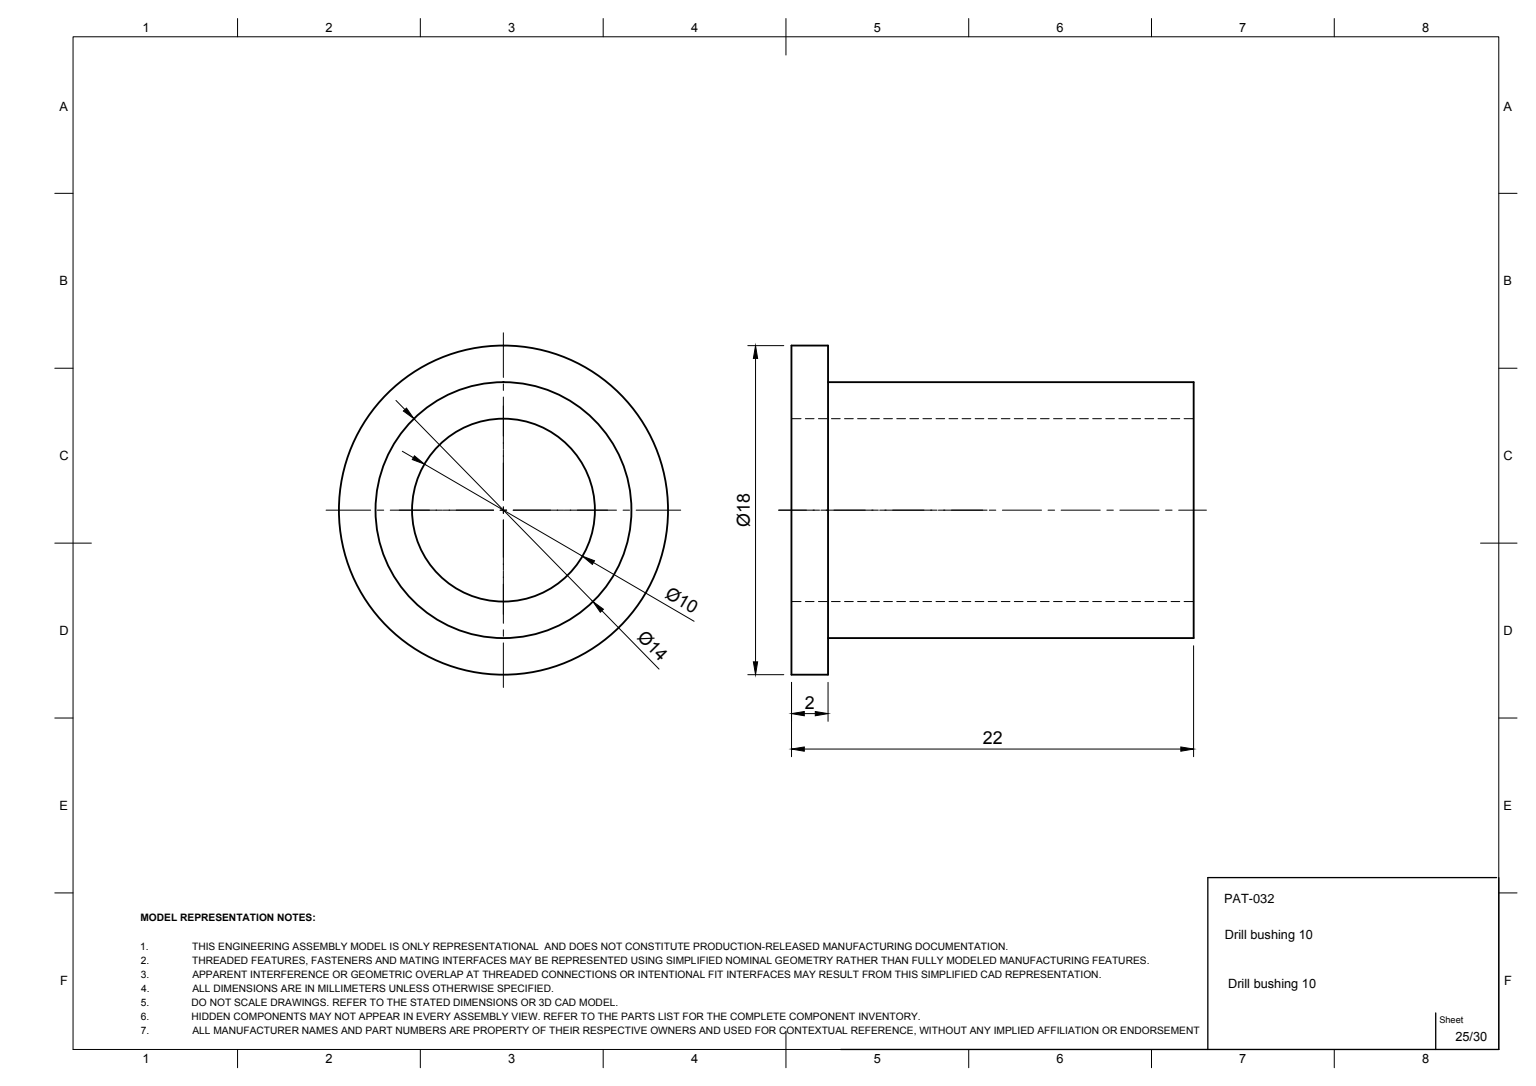
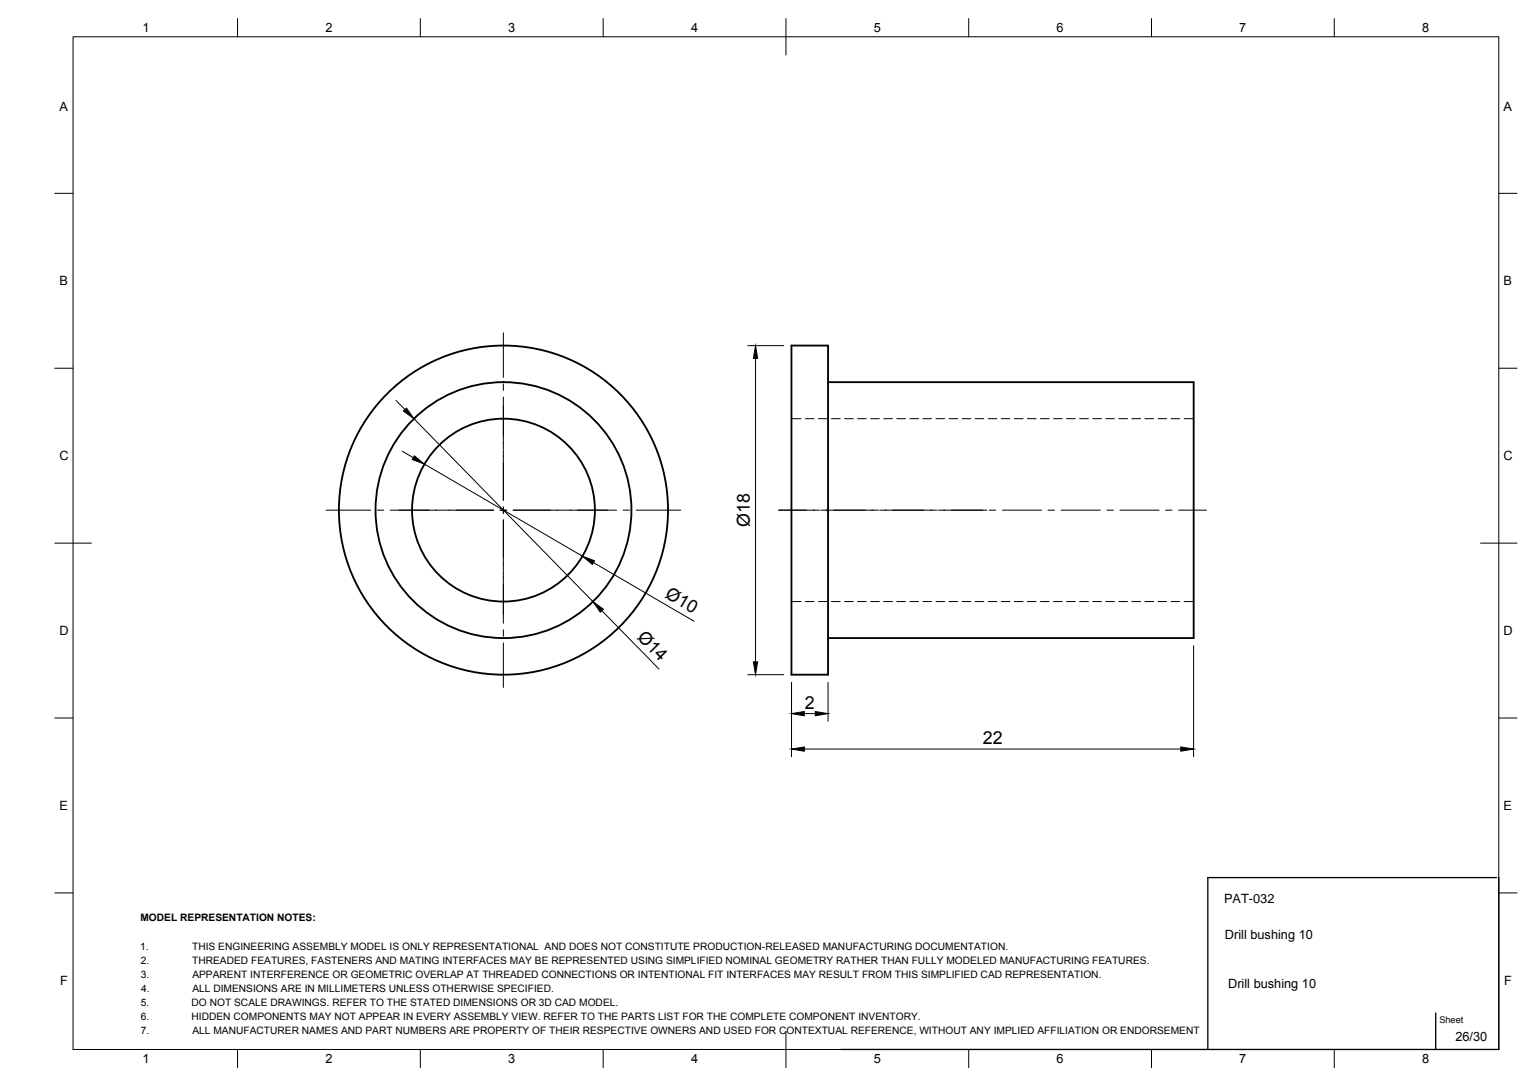
ISO-10303-21;
HEADER;
/* Generated by software containing ST-Developer
 * from STEP Tools, Inc. (www.steptools.com) 
 */

FILE_DESCRIPTION(
/* description */ ('Drill jig with bushing plate'),
/* implementation_level */ '2;1');

FILE_NAME(
/* name */ 'Drill bushing 10.step',
/* time_stamp */ '2026-10-27T10:51:08-07:00',
/* author */ (''),
/* organization */ (''),
/* preprocessor_version */ 'ST-DEVELOPER v20.2',
/* originating_system */ 'Autodesk Translation Framework v15.17.0.0',
/* authorisation */ '');

FILE_SCHEMA (('AUTOMOTIVE_DESIGN { 1 0 10303 214 3 1 1 }'));
ENDSEC;

DATA;
#10=MECHANICAL_DESIGN_GEOMETRIC_PRESENTATION_REPRESENTATION('',(#243),#6638);
#195=SHAPE_REPRESENTATION_RELATIONSHIP('SRR','None',#6760,#219);
#219=ADVANCED_BREP_SHAPE_REPRESENTATION('',(#265),#6633);
#243=STYLED_ITEM('',(#6929),#265);
#265=MANIFOLD_SOLID_BREP('Body1',#3612);
#361=FACE_BOUND('',#998,.T.);
#362=FACE_BOUND('',#1001,.T.);
#363=FACE_BOUND('',#1005,.T.);
#487=PLANE('',#4271);
#488=PLANE('',#4276);
#489=PLANE('',#4282);
#691=FACE_OUTER_BOUND('',#997,.T.);
#692=FACE_OUTER_BOUND('',#999,.T.);
#693=FACE_OUTER_BOUND('',#1000,.T.);
#694=FACE_OUTER_BOUND('',#1002,.T.);
#695=FACE_OUTER_BOUND('',#1003,.T.);
#696=FACE_OUTER_BOUND('',#1004,.T.);
#997=EDGE_LOOP('',(#3221));
#998=EDGE_LOOP('',(#3222));
#999=EDGE_LOOP('',(#3223,#3224,#3225,#3226));
#1000=EDGE_LOOP('',(#3227));
#1001=EDGE_LOOP('',(#3228));
#1002=EDGE_LOOP('',(#3229,#3230,#3231,#3232));
#1003=EDGE_LOOP('',(#3233,#3234,#3235,#3236));
#1004=EDGE_LOOP('',(#3237));
#1005=EDGE_LOOP('',(#3238));
#1272=LINE('',#6486,#1533);
#1273=LINE('',#6492,#1534);
#1274=LINE('',#6496,#1535);
#1533=VECTOR('',#5361,0.9);
#1534=VECTOR('',#5368,0.5);
#1535=VECTOR('',#5373,0.7);
#1700=CIRCLE('',#4272,0.9);
#1701=CIRCLE('',#4273,0.7);
#1702=CIRCLE('',#4275,0.9);
#1703=CIRCLE('',#4277,0.5);
#1704=CIRCLE('',#4279,0.5);
#1705=CIRCLE('',#4281,0.7);
#1980=VERTEX_POINT('',#6479);
#1981=VERTEX_POINT('',#6481);
#1982=VERTEX_POINT('',#6484);
#1983=VERTEX_POINT('',#6488);
#1984=VERTEX_POINT('',#6491);
#1985=VERTEX_POINT('',#6495);
#2398=EDGE_CURVE('',#1980,#1980,#1700,.T.);
#2399=EDGE_CURVE('',#1981,#1981,#1701,.T.);
#2400=EDGE_CURVE('',#1982,#1982,#1702,.T.);
#2401=EDGE_CURVE('',#1982,#1980,#1272,.T.);
#2402=EDGE_CURVE('',#1983,#1983,#1703,.T.);
#2403=EDGE_CURVE('',#1983,#1984,#1273,.T.);
#2404=EDGE_CURVE('',#1984,#1984,#1704,.T.);
#2405=EDGE_CURVE('',#1981,#1985,#1274,.T.);
#2406=EDGE_CURVE('',#1985,#1985,#1705,.T.);
#3221=ORIENTED_EDGE('',*,*,#2398,.F.);
#3222=ORIENTED_EDGE('',*,*,#2399,.T.);
#3223=ORIENTED_EDGE('',*,*,#2400,.F.);
#3224=ORIENTED_EDGE('',*,*,#2401,.T.);
#3225=ORIENTED_EDGE('',*,*,#2398,.T.);
#3226=ORIENTED_EDGE('',*,*,#2401,.F.);
#3227=ORIENTED_EDGE('',*,*,#2400,.T.);
#3228=ORIENTED_EDGE('',*,*,#2402,.T.);
#3229=ORIENTED_EDGE('',*,*,#2402,.F.);
#3230=ORIENTED_EDGE('',*,*,#2403,.T.);
#3231=ORIENTED_EDGE('',*,*,#2404,.T.);
#3232=ORIENTED_EDGE('',*,*,#2403,.F.);
#3233=ORIENTED_EDGE('',*,*,#2399,.F.);
#3234=ORIENTED_EDGE('',*,*,#2405,.T.);
#3235=ORIENTED_EDGE('',*,*,#2406,.T.);
#3236=ORIENTED_EDGE('',*,*,#2405,.F.);
#3237=ORIENTED_EDGE('',*,*,#2406,.F.);
#3238=ORIENTED_EDGE('',*,*,#2404,.F.);
#3366=CYLINDRICAL_SURFACE('',#4274,0.9);
#3367=CYLINDRICAL_SURFACE('',#4278,0.5);
#3368=CYLINDRICAL_SURFACE('',#4280,0.7);
#3566=ADVANCED_FACE('',(#691,#361),#487,.F.);
#3567=ADVANCED_FACE('',(#692),#3366,.T.);
#3568=ADVANCED_FACE('',(#693,#362),#488,.T.);
#3569=ADVANCED_FACE('',(#694),#3367,.F.);
#3570=ADVANCED_FACE('',(#695),#3368,.T.);
#3571=ADVANCED_FACE('',(#696,#363),#489,.F.);
#3612=CLOSED_SHELL('',(#3566,#3567,#3568,#3569,#3570,#3571));
#4270=AXIS2_PLACEMENT_3D('',#6477,#5349,#5350);
#4271=AXIS2_PLACEMENT_3D('',#6478,#5351,#5352);
#4272=AXIS2_PLACEMENT_3D('',#6480,#5353,#5354);
#4273=AXIS2_PLACEMENT_3D('',#6482,#5355,#5356);
#4274=AXIS2_PLACEMENT_3D('',#6483,#5357,#5358);
#4275=AXIS2_PLACEMENT_3D('',#6485,#5359,#5360);
#4276=AXIS2_PLACEMENT_3D('',#6487,#5362,#5363);
#4277=AXIS2_PLACEMENT_3D('',#6489,#5364,#5365);
#4278=AXIS2_PLACEMENT_3D('',#6490,#5366,#5367);
#4279=AXIS2_PLACEMENT_3D('',#6493,#5369,#5370);
#4280=AXIS2_PLACEMENT_3D('',#6494,#5371,#5372);
#4281=AXIS2_PLACEMENT_3D('',#6497,#5374,#5375);
#4282=AXIS2_PLACEMENT_3D('',#6498,#5376,#5377);
#5349=DIRECTION('axis',(0.,0.,1.));
#5350=DIRECTION('refdir',(1.,0.,0.));
#5351=DIRECTION('center_axis',(0.,0.,1.));
#5352=DIRECTION('ref_axis',(1.,0.,0.));
#5353=DIRECTION('center_axis',(0.,0.,1.));
#5354=DIRECTION('ref_axis',(1.,0.,0.));
#5355=DIRECTION('center_axis',(0.,0.,1.));
#5356=DIRECTION('ref_axis',(1.,0.,0.));
#5357=DIRECTION('center_axis',(0.,0.,1.));
#5358=DIRECTION('ref_axis',(1.,0.,0.));
#5359=DIRECTION('center_axis',(0.,0.,1.));
#5360=DIRECTION('ref_axis',(1.,0.,0.));
#5361=DIRECTION('',(0.,0.,-1.));
#5362=DIRECTION('center_axis',(0.,0.,1.));
#5363=DIRECTION('ref_axis',(1.,0.,0.));
#5364=DIRECTION('center_axis',(0.,0.,-1.));
#5365=DIRECTION('ref_axis',(1.,0.,0.));
#5366=DIRECTION('center_axis',(0.,0.,1.));
#5367=DIRECTION('ref_axis',(1.,0.,0.));
#5368=DIRECTION('',(0.,0.,-1.));
#5369=DIRECTION('center_axis',(0.,0.,-1.));
#5370=DIRECTION('ref_axis',(1.,0.,0.));
#5371=DIRECTION('center_axis',(0.,0.,1.));
#5372=DIRECTION('ref_axis',(1.,0.,0.));
#5373=DIRECTION('',(0.,0.,-1.));
#5374=DIRECTION('center_axis',(0.,0.,1.));
#5375=DIRECTION('ref_axis',(1.,0.,0.));
#5376=DIRECTION('center_axis',(0.,0.,1.));
#5377=DIRECTION('ref_axis',(1.,0.,0.));
#6477=CARTESIAN_POINT('',(0.,0.,0.));
#6478=CARTESIAN_POINT('Origin',(2.,-1.,4.5));
#6479=CARTESIAN_POINT('',(1.1,-1.,4.5));
#6480=CARTESIAN_POINT('Origin',(2.,-1.,4.5));
#6481=CARTESIAN_POINT('',(1.3,-1.,4.5));
#6482=CARTESIAN_POINT('Origin',(2.,-1.,4.5));
#6483=CARTESIAN_POINT('Origin',(2.,-1.,4.5));
#6484=CARTESIAN_POINT('',(1.1,-1.,4.7));
#6485=CARTESIAN_POINT('Origin',(2.,-1.,4.7));
#6486=CARTESIAN_POINT('',(1.1,-1.,4.5));
#6487=CARTESIAN_POINT('Origin',(2.,-1.,4.7));
#6488=CARTESIAN_POINT('',(1.5,-1.,4.7));
#6489=CARTESIAN_POINT('Origin',(2.,-1.,4.7));
#6490=CARTESIAN_POINT('Origin',(2.,-1.,2.5));
#6491=CARTESIAN_POINT('',(1.5,-1.,2.5));
#6492=CARTESIAN_POINT('',(1.5,-1.,2.5));
#6493=CARTESIAN_POINT('Origin',(2.,-1.,2.5));
#6494=CARTESIAN_POINT('Origin',(2.,-1.,2.5));
#6495=CARTESIAN_POINT('',(1.3,-1.,2.5));
#6496=CARTESIAN_POINT('',(1.3,-1.,2.5));
#6497=CARTESIAN_POINT('Origin',(2.,-1.,2.5));
#6498=CARTESIAN_POINT('Origin',(2.,-1.,2.5));
#6604=UNCERTAINTY_MEASURE_WITH_UNIT(LENGTH_MEASURE(0.001),#6639,
'DISTANCE_ACCURACY_VALUE',
'Maximum model space distance between geometric entities at asserted c
onnectivities');
#6609=UNCERTAINTY_MEASURE_WITH_UNIT(LENGTH_MEASURE(0.001),#6639,
'DISTANCE_ACCURACY_VALUE',
'Maximum model space distance between geometric entities at asserted c
onnectivities');
#6633=(
GEOMETRIC_REPRESENTATION_CONTEXT(3)
GLOBAL_UNCERTAINTY_ASSIGNED_CONTEXT((#6604))
GLOBAL_UNIT_ASSIGNED_CONTEXT((#6639,#6641,#6642))
REPRESENTATION_CONTEXT('','3D')
);
#6638=(
GEOMETRIC_REPRESENTATION_CONTEXT(3)
GLOBAL_UNCERTAINTY_ASSIGNED_CONTEXT((#6609))
GLOBAL_UNIT_ASSIGNED_CONTEXT((#6639,#6641,#6642))
REPRESENTATION_CONTEXT('','3D')
);
#6639=(
LENGTH_UNIT()
NAMED_UNIT(*)
SI_UNIT(.CENTI.,.METRE.)
);
#6641=(
NAMED_UNIT(*)
PLANE_ANGLE_UNIT()
SI_UNIT($,.RADIAN.)
);
#6642=(
NAMED_UNIT(*)
SI_UNIT($,.STERADIAN.)
SOLID_ANGLE_UNIT()
);
#6666=SHAPE_DEFINITION_REPRESENTATION(#6722,#6760);
#6722=PRODUCT_DEFINITION_SHAPE('',$,#6789);
#6760=SHAPE_REPRESENTATION('',(#4270),#6633);
#6765=PRODUCT_DEFINITION_CONTEXT('part definition',#6851,'design');
#6789=PRODUCT_DEFINITION('Drill bushing 10','Drill bushing 10',#6817,#6765);
#6817=PRODUCT_DEFINITION_FORMATION('',$,#6876);
#6851=APPLICATION_CONTEXT(
'Core Data for Automotive Mechanical Design Process');
#6852=PRODUCT_CONTEXT('part definition',#6851,'mechanical');
#6876=PRODUCT('Drill bushing 10','Drill bushing 10','Drill bushing 10',
(#6852));
#6923=COLOUR_RGB('Light Blue',0.38,0.62,0.78);
#6924=FILL_AREA_STYLE_COLOUR('',#6923);
#6925=FILL_AREA_STYLE('',(#6924));
#6926=SURFACE_STYLE_FILL_AREA(#6925);
#6927=SURFACE_SIDE_STYLE('',(#6926));
#6928=SURFACE_STYLE_USAGE(.BOTH.,#6927);
#6929=PRESENTATION_STYLE_ASSIGNMENT((#6928));
ENDSEC;
END-ISO-10303-21;
